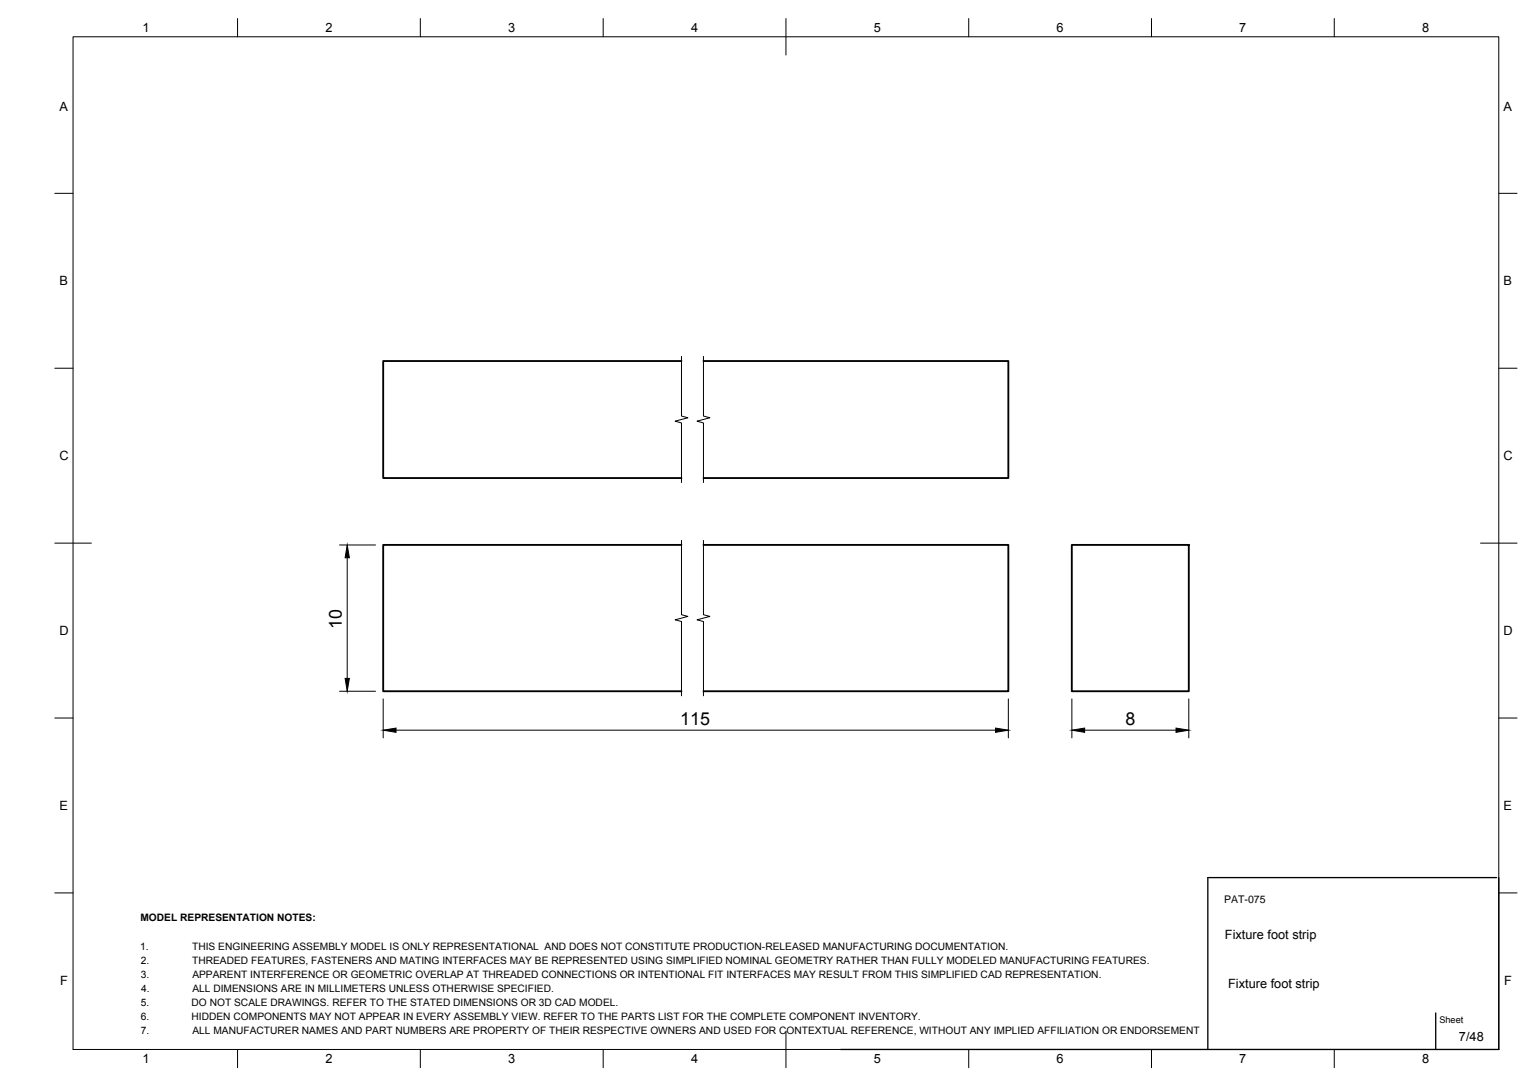
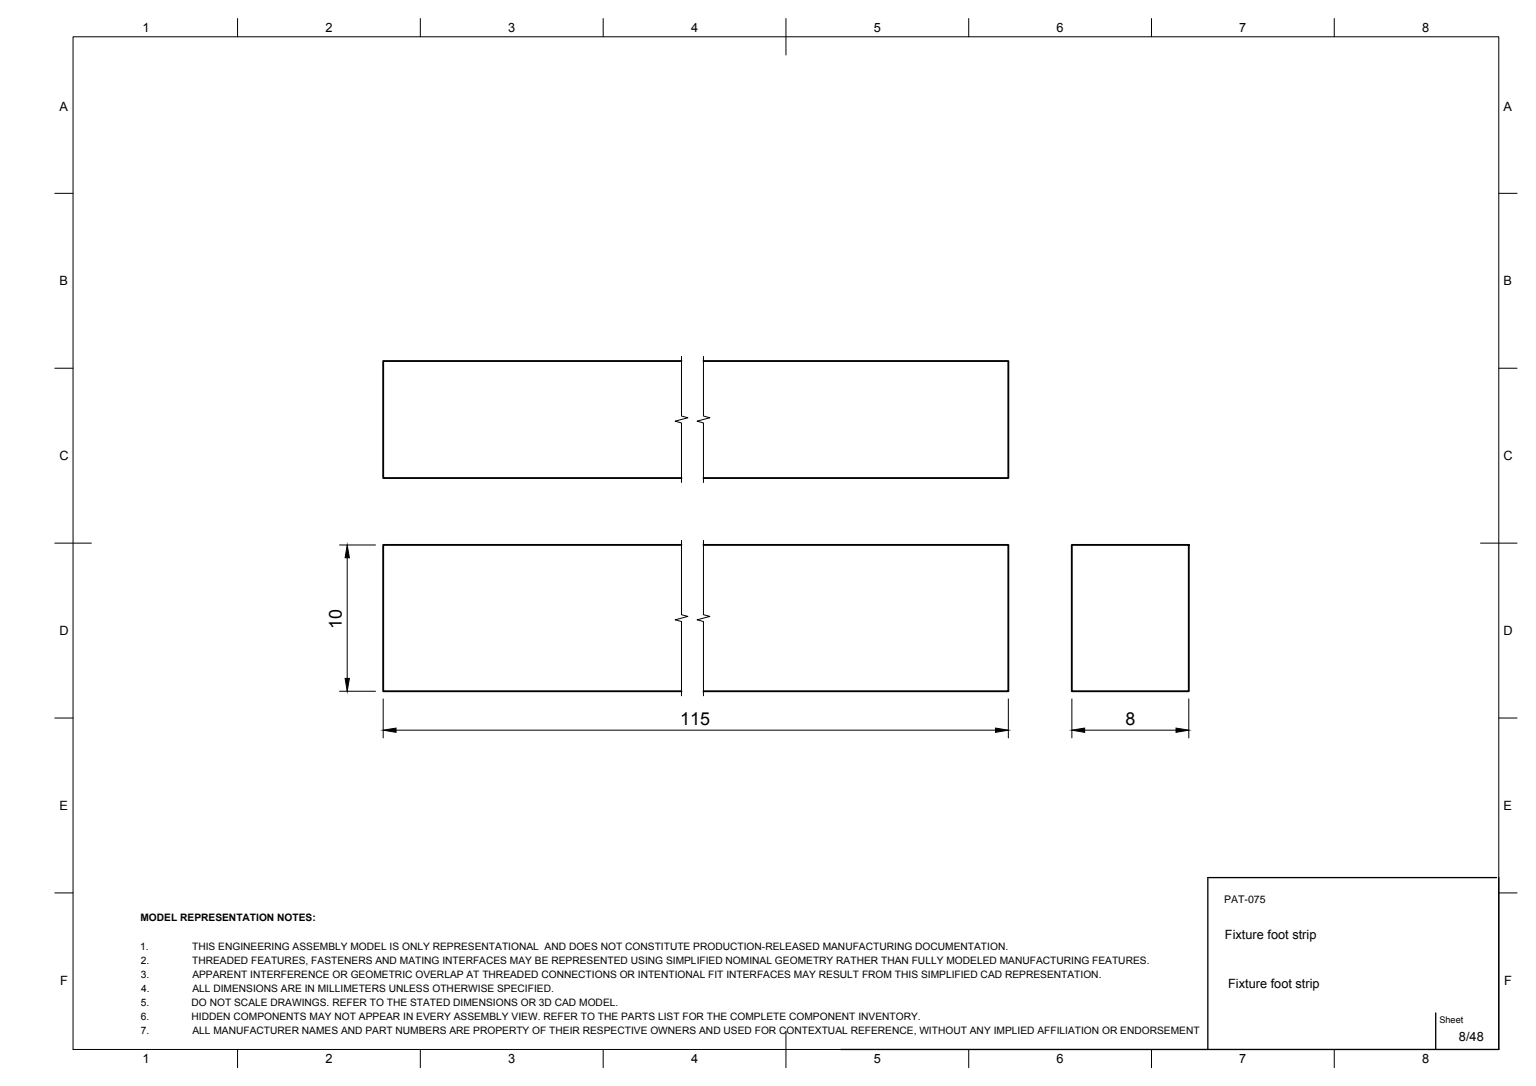
ISO-10303-21;
HEADER;
/* Generated by software containing ST-Developer
 * from STEP Tools, Inc. (www.steptools.com) 
 */

FILE_DESCRIPTION(
/* description */ ('Over-Centre Plunger Toggle Clamp on Slotted Fixture Frame'),
/* implementation_level */ '2;1');

FILE_NAME(
/* name */ 
'Fixture foot strip.step',
/* time_stamp */ '2026-10-28T03:23:24-07:00',
/* author */ (''),
/* organization */ (''),
/* preprocessor_version */ 'ST-DEVELOPER v20.2',
/* originating_system */ 'Autodesk Translation Framework v15.17.0.0',
/* authorisation */ '');

FILE_SCHEMA (('AUTOMOTIVE_DESIGN { 1 0 10303 214 3 1 1 }'));
ENDSEC;

DATA;
#10=MECHANICAL_DESIGN_GEOMETRIC_PRESENTATION_REPRESENTATION('',(#515),#15212);
#431=SHAPE_REPRESENTATION_RELATIONSHIP('SRR','None',#15405,#473);
#473=ADVANCED_BREP_SHAPE_REPRESENTATION('',(#566),#15167);
#515=STYLED_ITEM('',(#15733),#566);
#566=MANIFOLD_SOLID_BREP('Body1',#8247);
#795=PLANE('',#8828);
#796=PLANE('',#8829);
#797=PLANE('',#8830);
#798=PLANE('',#8831);
#799=PLANE('',#8832);
#800=PLANE('',#8833);
#1115=FACE_OUTER_BOUND('',#1633,.T.);
#1116=FACE_OUTER_BOUND('',#1634,.T.);
#1117=FACE_OUTER_BOUND('',#1635,.T.);
#1118=FACE_OUTER_BOUND('',#1636,.T.);
#1119=FACE_OUTER_BOUND('',#1637,.T.);
#1120=FACE_OUTER_BOUND('',#1638,.T.);
#1633=EDGE_LOOP('',(#5713,#5714,#5715,#5716));
#1634=EDGE_LOOP('',(#5717,#5718,#5719,#5720));
#1635=EDGE_LOOP('',(#5721,#5722,#5723,#5724));
#1636=EDGE_LOOP('',(#5725,#5726,#5727,#5728));
#1637=EDGE_LOOP('',(#5729,#5730,#5731,#5732));
#1638=EDGE_LOOP('',(#5733,#5734,#5735,#5736));
#2271=LINE('',#12522,#2901);
#2272=LINE('',#12524,#2902);
#2273=LINE('',#12526,#2903);
#2274=LINE('',#12527,#2904);
#2275=LINE('',#12530,#2905);
#2276=LINE('',#12532,#2906);
#2277=LINE('',#12533,#2907);
#2278=LINE('',#12536,#2908);
#2279=LINE('',#12538,#2909);
#2280=LINE('',#12539,#2910);
#2281=LINE('',#12541,#2911);
#2282=LINE('',#12542,#2912);
#2901=VECTOR('',#9926,1.);
#2902=VECTOR('',#9927,1.);
#2903=VECTOR('',#9928,1.);
#2904=VECTOR('',#9929,1.);
#2905=VECTOR('',#9932,1.);
#2906=VECTOR('',#9933,1.);
#2907=VECTOR('',#9934,1.);
#2908=VECTOR('',#9937,1.);
#2909=VECTOR('',#9938,1.);
#2910=VECTOR('',#9939,1.);
#2911=VECTOR('',#9942,1.);
#2912=VECTOR('',#9943,1.);
#3907=VERTEX_POINT('',#12520);
#3908=VERTEX_POINT('',#12521);
#3909=VERTEX_POINT('',#12523);
#3910=VERTEX_POINT('',#12525);
#3911=VERTEX_POINT('',#12529);
#3912=VERTEX_POINT('',#12531);
#3913=VERTEX_POINT('',#12535);
#3914=VERTEX_POINT('',#12537);
#4617=EDGE_CURVE('',#3907,#3908,#2271,.T.);
#4618=EDGE_CURVE('',#3908,#3909,#2272,.T.);
#4619=EDGE_CURVE('',#3910,#3909,#2273,.T.);
#4620=EDGE_CURVE('',#3907,#3910,#2274,.T.);
#4621=EDGE_CURVE('',#3911,#3907,#2275,.T.);
#4622=EDGE_CURVE('',#3912,#3910,#2276,.T.);
#4623=EDGE_CURVE('',#3911,#3912,#2277,.T.);
#4624=EDGE_CURVE('',#3913,#3911,#2278,.T.);
#4625=EDGE_CURVE('',#3914,#3912,#2279,.T.);
#4626=EDGE_CURVE('',#3913,#3914,#2280,.T.);
#4627=EDGE_CURVE('',#3908,#3913,#2281,.T.);
#4628=EDGE_CURVE('',#3909,#3914,#2282,.T.);
#5713=ORIENTED_EDGE('',*,*,#4617,.T.);
#5714=ORIENTED_EDGE('',*,*,#4618,.T.);
#5715=ORIENTED_EDGE('',*,*,#4619,.F.);
#5716=ORIENTED_EDGE('',*,*,#4620,.F.);
#5717=ORIENTED_EDGE('',*,*,#4621,.T.);
#5718=ORIENTED_EDGE('',*,*,#4620,.T.);
#5719=ORIENTED_EDGE('',*,*,#4622,.F.);
#5720=ORIENTED_EDGE('',*,*,#4623,.F.);
#5721=ORIENTED_EDGE('',*,*,#4624,.T.);
#5722=ORIENTED_EDGE('',*,*,#4623,.T.);
#5723=ORIENTED_EDGE('',*,*,#4625,.F.);
#5724=ORIENTED_EDGE('',*,*,#4626,.F.);
#5725=ORIENTED_EDGE('',*,*,#4627,.T.);
#5726=ORIENTED_EDGE('',*,*,#4626,.T.);
#5727=ORIENTED_EDGE('',*,*,#4628,.F.);
#5728=ORIENTED_EDGE('',*,*,#4618,.F.);
#5729=ORIENTED_EDGE('',*,*,#4628,.T.);
#5730=ORIENTED_EDGE('',*,*,#4625,.T.);
#5731=ORIENTED_EDGE('',*,*,#4622,.T.);
#5732=ORIENTED_EDGE('',*,*,#4619,.T.);
#5733=ORIENTED_EDGE('',*,*,#4627,.F.);
#5734=ORIENTED_EDGE('',*,*,#4617,.F.);
#5735=ORIENTED_EDGE('',*,*,#4621,.F.);
#5736=ORIENTED_EDGE('',*,*,#4624,.F.);
#7787=ADVANCED_FACE('',(#1115),#795,.T.);
#7788=ADVANCED_FACE('',(#1116),#796,.T.);
#7789=ADVANCED_FACE('',(#1117),#797,.T.);
#7790=ADVANCED_FACE('',(#1118),#798,.T.);
#7791=ADVANCED_FACE('',(#1119),#799,.T.);
#7792=ADVANCED_FACE('',(#1120),#800,.F.);
#8247=CLOSED_SHELL('',(#7787,#7788,#7789,#7790,#7791,#7792));
#8827=AXIS2_PLACEMENT_3D('',#12518,#9922,#9923);
#8828=AXIS2_PLACEMENT_3D('',#12519,#9924,#9925);
#8829=AXIS2_PLACEMENT_3D('',#12528,#9930,#9931);
#8830=AXIS2_PLACEMENT_3D('',#12534,#9935,#9936);
#8831=AXIS2_PLACEMENT_3D('',#12540,#9940,#9941);
#8832=AXIS2_PLACEMENT_3D('',#12543,#9944,#9945);
#8833=AXIS2_PLACEMENT_3D('',#12544,#9946,#9947);
#9922=DIRECTION('axis',(0.,0.,1.));
#9923=DIRECTION('refdir',(1.,0.,0.));
#9924=DIRECTION('center_axis',(0.,1.,0.));
#9925=DIRECTION('ref_axis',(-1.,0.,0.));
#9926=DIRECTION('',(-1.,0.,0.));
#9927=DIRECTION('',(0.,0.,1.));
#9928=DIRECTION('',(-1.,0.,0.));
#9929=DIRECTION('',(0.,0.,1.));
#9930=DIRECTION('center_axis',(1.,0.,0.));
#9931=DIRECTION('ref_axis',(0.,1.,0.));
#9932=DIRECTION('',(0.,1.,0.));
#9933=DIRECTION('',(0.,1.,0.));
#9934=DIRECTION('',(0.,0.,1.));
#9935=DIRECTION('center_axis',(0.,-1.,0.));
#9936=DIRECTION('ref_axis',(1.,0.,0.));
#9937=DIRECTION('',(1.,0.,0.));
#9938=DIRECTION('',(1.,0.,0.));
#9939=DIRECTION('',(0.,0.,1.));
#9940=DIRECTION('center_axis',(-1.,0.,0.));
#9941=DIRECTION('ref_axis',(0.,-1.,0.));
#9942=DIRECTION('',(0.,-1.,0.));
#9943=DIRECTION('',(0.,-1.,0.));
#9944=DIRECTION('center_axis',(0.,0.,1.));
#9945=DIRECTION('ref_axis',(1.,0.,0.));
#9946=DIRECTION('center_axis',(0.,0.,1.));
#9947=DIRECTION('ref_axis',(1.,0.,0.));
#12518=CARTESIAN_POINT('',(0.,0.,0.));
#12519=CARTESIAN_POINT('Origin',(-8.5,4.5,-3.6));
#12520=CARTESIAN_POINT('',(-8.5,4.5,-3.6));
#12521=CARTESIAN_POINT('',(-9.5,4.5,-3.6));
#12522=CARTESIAN_POINT('',(-8.5,4.5,-3.6));
#12523=CARTESIAN_POINT('',(-9.5,4.5,-2.8));
#12524=CARTESIAN_POINT('',(-9.5,4.5,-3.6));
#12525=CARTESIAN_POINT('',(-8.5,4.5,-2.8));
#12526=CARTESIAN_POINT('',(-8.5,4.5,-2.8));
#12527=CARTESIAN_POINT('',(-8.5,4.5,-3.6));
#12528=CARTESIAN_POINT('Origin',(-8.5,-7.,-3.6));
#12529=CARTESIAN_POINT('',(-8.5,-7.,-3.6));
#12530=CARTESIAN_POINT('',(-8.5,-7.,-3.6));
#12531=CARTESIAN_POINT('',(-8.5,-7.,-2.8));
#12532=CARTESIAN_POINT('',(-8.5,-7.,-2.8));
#12533=CARTESIAN_POINT('',(-8.5,-7.,-3.6));
#12534=CARTESIAN_POINT('Origin',(-9.5,-7.,-3.6));
#12535=CARTESIAN_POINT('',(-9.5,-7.,-3.6));
#12536=CARTESIAN_POINT('',(-9.5,-7.,-3.6));
#12537=CARTESIAN_POINT('',(-9.5,-7.,-2.8));
#12538=CARTESIAN_POINT('',(-9.5,-7.,-2.8));
#12539=CARTESIAN_POINT('',(-9.5,-7.,-3.6));
#12540=CARTESIAN_POINT('Origin',(-9.5,4.5,-3.6));
#12541=CARTESIAN_POINT('',(-9.5,4.5,-3.6));
#12542=CARTESIAN_POINT('',(-9.5,4.5,-2.8));
#12543=CARTESIAN_POINT('Origin',(-9.,-1.25,-2.8));
#12544=CARTESIAN_POINT('Origin',(-9.,-1.25,-3.6));
#15117=UNCERTAINTY_MEASURE_WITH_UNIT(LENGTH_MEASURE(0.001),#15213,
'DISTANCE_ACCURACY_VALUE',
'Maximum model space distance between geometric entities at asserted c
onnectivities');
#15162=UNCERTAINTY_MEASURE_WITH_UNIT(LENGTH_MEASURE(0.001),#15213,
'DISTANCE_ACCURACY_VALUE',
'Maximum model space distance between geometric entities at asserted c
onnectivities');
#15167=(
GEOMETRIC_REPRESENTATION_CONTEXT(3)
GLOBAL_UNCERTAINTY_ASSIGNED_CONTEXT((#15117))
GLOBAL_UNIT_ASSIGNED_CONTEXT((#15213,#15215,#15216))
REPRESENTATION_CONTEXT('','3D')
);
#15212=(
GEOMETRIC_REPRESENTATION_CONTEXT(3)
GLOBAL_UNCERTAINTY_ASSIGNED_CONTEXT((#15162))
GLOBAL_UNIT_ASSIGNED_CONTEXT((#15213,#15215,#15216))
REPRESENTATION_CONTEXT('','3D')
);
#15213=(
LENGTH_UNIT()
NAMED_UNIT(*)
SI_UNIT(.CENTI.,.METRE.)
);
#15215=(
NAMED_UNIT(*)
PLANE_ANGLE_UNIT()
SI_UNIT($,.RADIAN.)
);
#15216=(
NAMED_UNIT(*)
SI_UNIT($,.STERADIAN.)
SOLID_ANGLE_UNIT()
);
#15221=SHAPE_DEFINITION_REPRESENTATION(#15270,#15405);
#15270=PRODUCT_DEFINITION_SHAPE('',$,#15455);
#15405=SHAPE_REPRESENTATION('',(#8827),#15167);
#15450=PRODUCT_DEFINITION_CONTEXT('part definition',#15599,'design');
#15455=PRODUCT_DEFINITION('Fixture foot strip','Fixture foot strip',#15504,
#15450);
#15504=PRODUCT_DEFINITION_FORMATION('',$,#15605);
#15599=APPLICATION_CONTEXT(
'Core Data for Automotive Mechanical Design Process');
#15600=PRODUCT_CONTEXT('part definition',#15599,'mechanical');
#15605=PRODUCT('Fixture foot strip','Fixture foot strip',
'Fixture foot strip',(#15600));
#15727=COLOUR_RGB('Off White',0.89,0.88,0.83);
#15728=FILL_AREA_STYLE_COLOUR('',#15727);
#15729=FILL_AREA_STYLE('',(#15728));
#15730=SURFACE_STYLE_FILL_AREA(#15729);
#15731=SURFACE_SIDE_STYLE('',(#15730));
#15732=SURFACE_STYLE_USAGE(.BOTH.,#15731);
#15733=PRESENTATION_STYLE_ASSIGNMENT((#15732));
ENDSEC;
END-ISO-10303-21;
